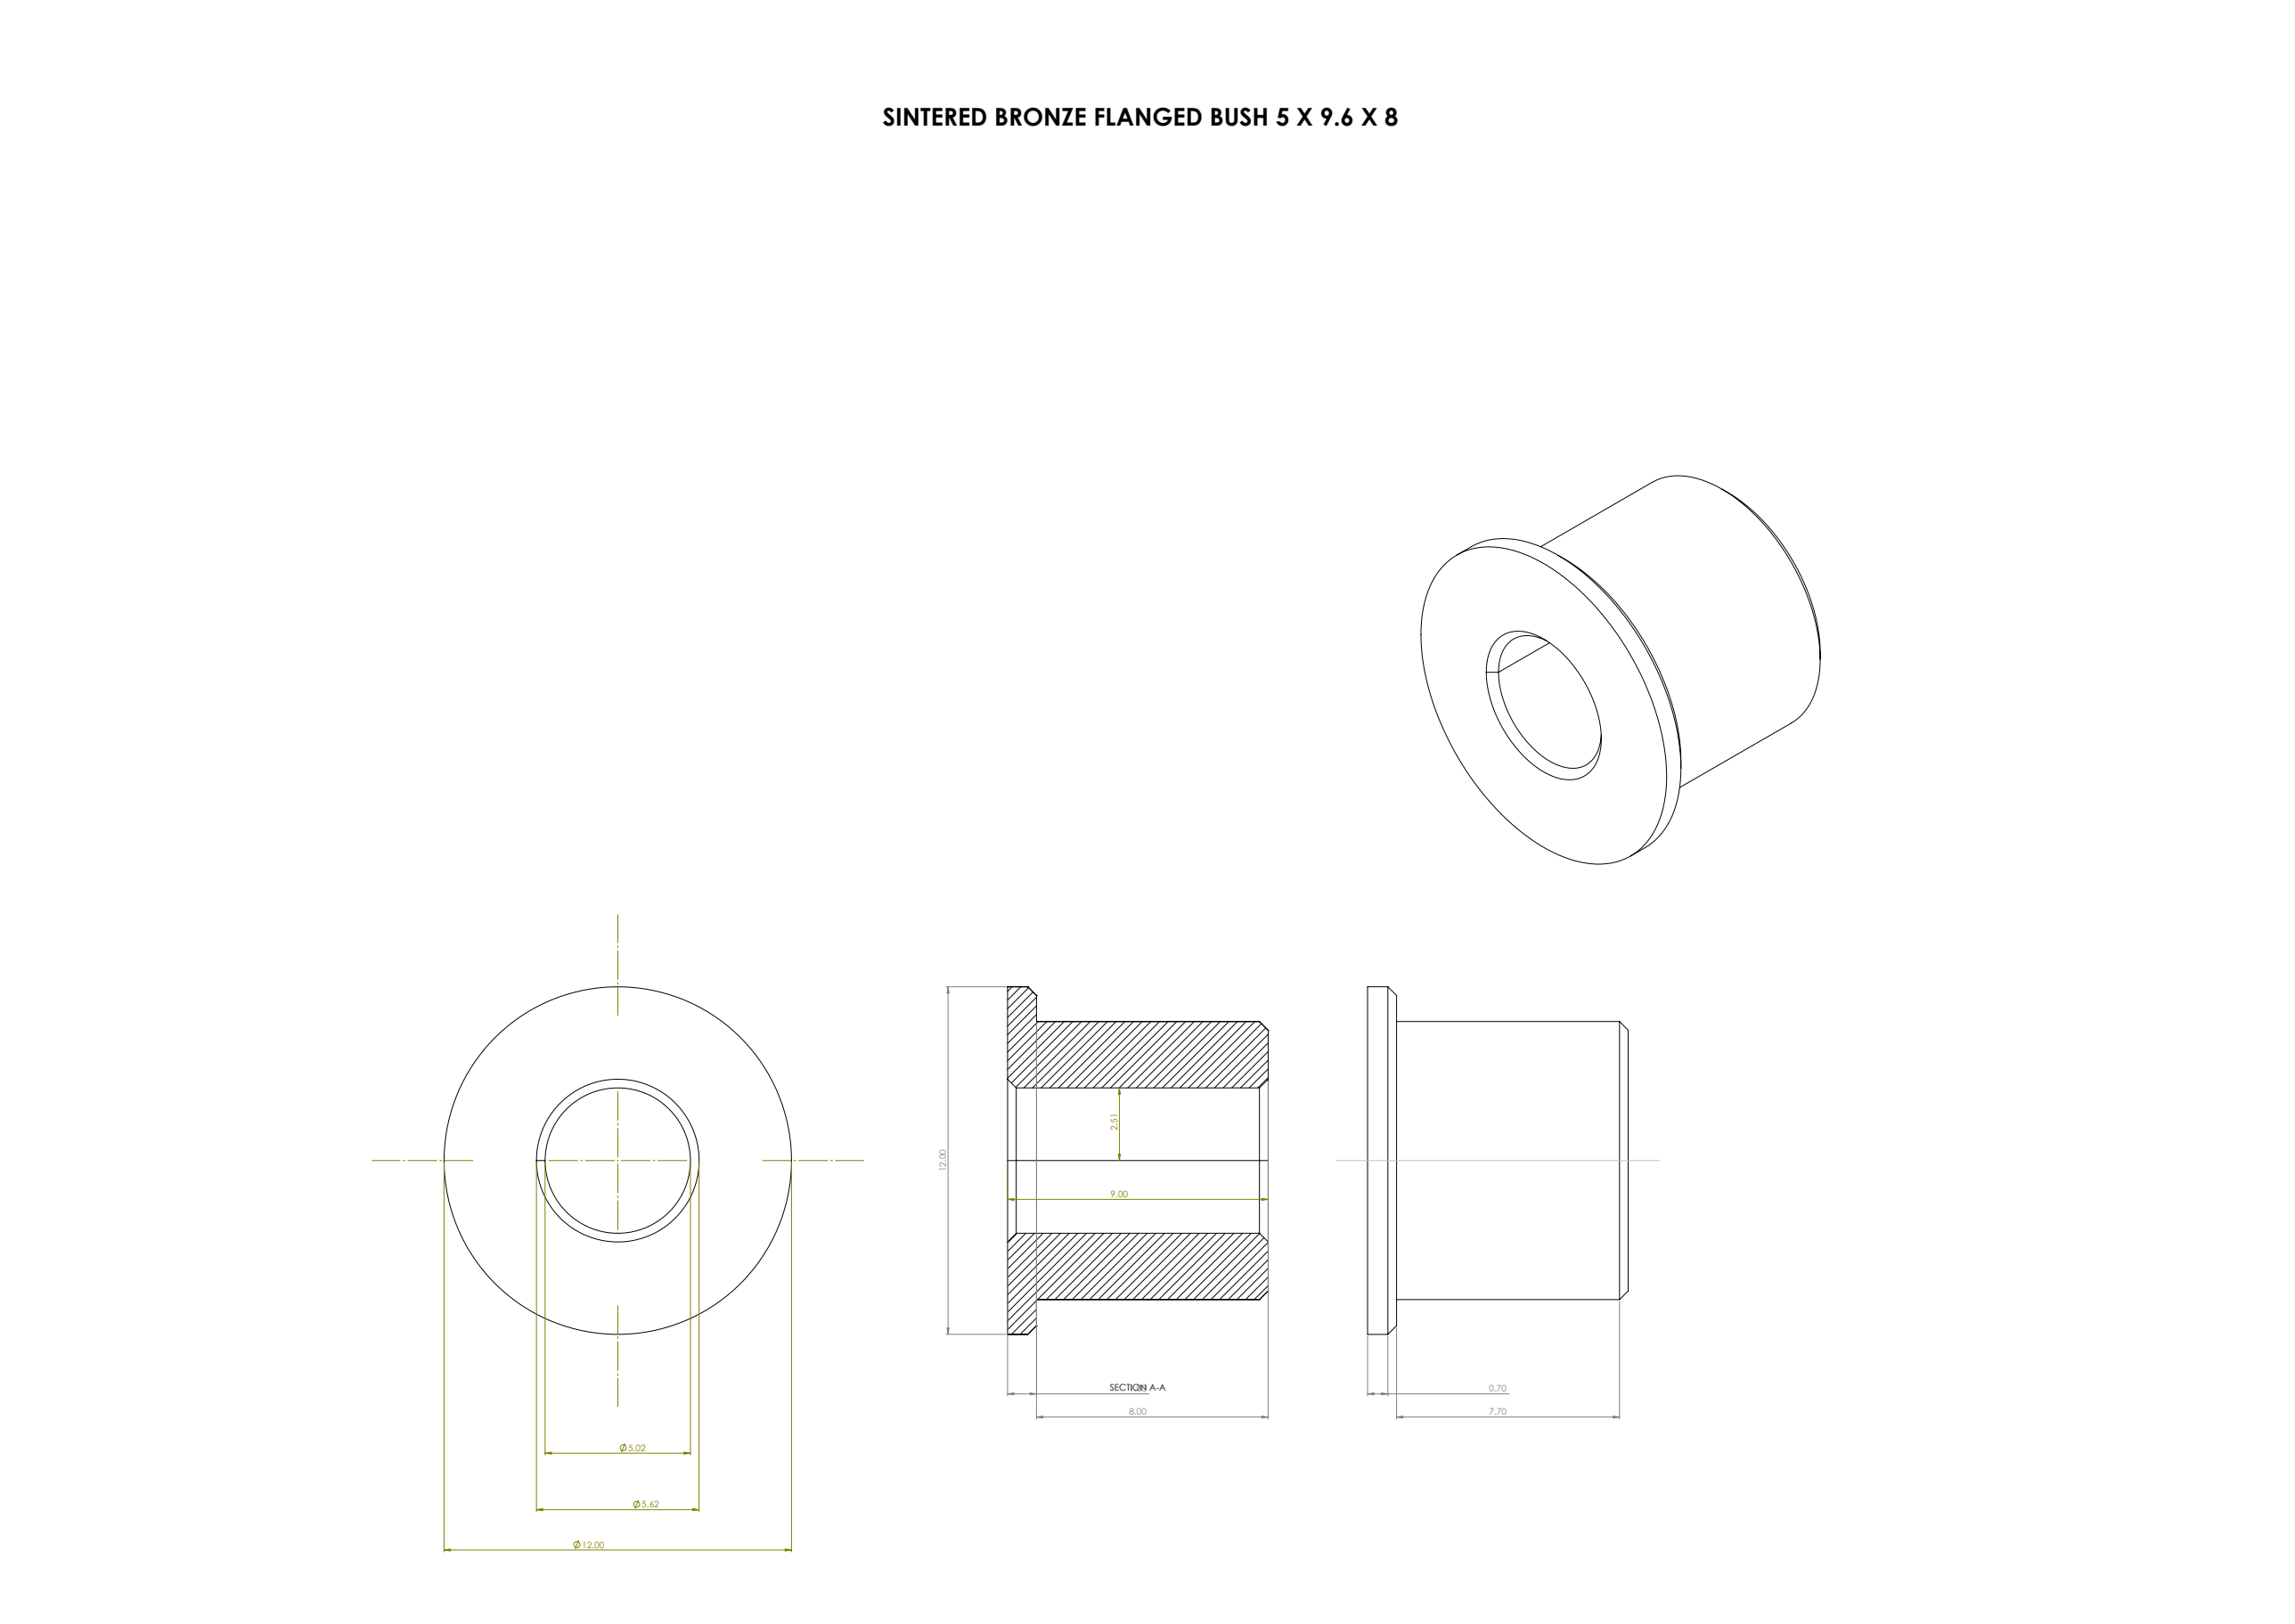
ISO-10303-21;
HEADER;
/* Generated by software containing ST-Developer
 * from STEP Tools, Inc. (www.steptools.com) 
 */

FILE_DESCRIPTION(
/* description */ (''),
/* implementation_level */ '2;1');

FILE_NAME(
/* name */ 'Sintered Bronze Flanged Bush 5 x 9.6 x 8.step',
/* time_stamp */ '2026-10-05T09:57:53+05:00',
/* author */ (''),
/* organization */ (''),
/* preprocessor_version */ 'ST-DEVELOPER v20.2',
/* originating_system */ 'Autodesk Translation Framework v15.15.0.0',
/* authorisation */ '');

FILE_SCHEMA (('AUTOMOTIVE_DESIGN { 1 0 10303 214 3 1 1 }'));
ENDSEC;

DATA;
#10=MECHANICAL_DESIGN_GEOMETRIC_PRESENTATION_REPRESENTATION('',(#557),#113984);
#521=SHAPE_REPRESENTATION_RELATIONSHIP('SRR','None',#114058,#539);
#539=ADVANCED_BREP_SHAPE_REPRESENTATION('',(#575),#113972);
#557=STYLED_ITEM('',(#114296),#575);
#575=MANIFOLD_SOLID_BREP('Sintered Bronze Flanged Bush 5 x 9.6 x 8',#60398);
#700=CYLINDRICAL_SURFACE('',#62383,4.8);
#701=CYLINDRICAL_SURFACE('',#62389,6.);
#702=CYLINDRICAL_SURFACE('',#62395,2.51000000000001);
#922=CONICAL_SURFACE('',#62376,2.66000000000002,0.785398163397434);
#923=CONICAL_SURFACE('',#62381,4.65,0.785398163397463);
#924=CONICAL_SURFACE('',#62387,5.85000000000001,0.785398163397434);
#925=CONICAL_SURFACE('',#62393,2.66000000000002,0.785398163397434);
#1234=CIRCLE('',#62377,2.51000000000001);
#1235=CIRCLE('',#62378,2.81000000000001);
#1236=CIRCLE('',#62380,4.49999999999999);
#1237=CIRCLE('',#62382,4.8);
#1238=CIRCLE('',#62384,4.8);
#1239=CIRCLE('',#62386,5.7);
#1240=CIRCLE('',#62388,6.);
#1241=CIRCLE('',#62390,6.);
#1242=CIRCLE('',#62392,2.81000000000001);
#1243=CIRCLE('',#62394,2.51000000000001);
#1838=FACE_BOUND('',#9788,.T.);
#1839=FACE_BOUND('',#9792,.T.);
#1840=FACE_BOUND('',#9796,.T.);
#3183=PLANE('',#62379);
#3184=PLANE('',#62385);
#3185=PLANE('',#62391);
#6223=FACE_OUTER_BOUND('',#9786,.T.);
#6224=FACE_OUTER_BOUND('',#9787,.T.);
#6225=FACE_OUTER_BOUND('',#9789,.T.);
#6226=FACE_OUTER_BOUND('',#9790,.T.);
#6227=FACE_OUTER_BOUND('',#9791,.T.);
#6228=FACE_OUTER_BOUND('',#9793,.T.);
#6229=FACE_OUTER_BOUND('',#9794,.T.);
#6230=FACE_OUTER_BOUND('',#9795,.T.);
#6231=FACE_OUTER_BOUND('',#9797,.T.);
#6232=FACE_OUTER_BOUND('',#9798,.T.);
#9786=EDGE_LOOP('',(#50399,#50400,#50401,#50402));
#9787=EDGE_LOOP('',(#50403));
#9788=EDGE_LOOP('',(#50404));
#9789=EDGE_LOOP('',(#50405,#50406,#50407,#50408));
#9790=EDGE_LOOP('',(#50409,#50410,#50411,#50412));
#9791=EDGE_LOOP('',(#50413));
#9792=EDGE_LOOP('',(#50414));
#9793=EDGE_LOOP('',(#50415,#50416,#50417,#50418));
#9794=EDGE_LOOP('',(#50419,#50420,#50421,#50422));
#9795=EDGE_LOOP('',(#50423));
#9796=EDGE_LOOP('',(#50424));
#9797=EDGE_LOOP('',(#50425,#50426,#50427,#50428));
#9798=EDGE_LOOP('',(#50429,#50430,#50431,#50432));
#14630=LINE('',#98912,#20664);
#14631=LINE('',#98920,#20665);
#14632=LINE('',#98924,#20666);
#14633=LINE('',#98931,#20667);
#14634=LINE('',#98935,#20668);
#14635=LINE('',#98941,#20669);
#14636=LINE('',#98944,#20670);
#20664=VECTOR('',#71068,2.66000000000002);
#20665=VECTOR('',#71079,4.65);
#20666=VECTOR('',#71084,4.8);
#20667=VECTOR('',#71093,5.85000000000001);
#20668=VECTOR('',#71098,6.);
#20669=VECTOR('',#71105,2.66000000000002);
#20670=VECTOR('',#71110,2.51000000000001);
#28381=VERTEX_POINT('',#98909);
#28382=VERTEX_POINT('',#98911);
#28383=VERTEX_POINT('',#98915);
#28384=VERTEX_POINT('',#98918);
#28385=VERTEX_POINT('',#98922);
#28386=VERTEX_POINT('',#98926);
#28387=VERTEX_POINT('',#98929);
#28388=VERTEX_POINT('',#98933);
#28389=VERTEX_POINT('',#98937);
#28390=VERTEX_POINT('',#98940);
#36032=EDGE_CURVE('',#28381,#28381,#1234,.T.);
#36033=EDGE_CURVE('',#28381,#28382,#14630,.T.);
#36034=EDGE_CURVE('',#28382,#28382,#1235,.T.);
#36035=EDGE_CURVE('',#28383,#28383,#1236,.T.);
#36036=EDGE_CURVE('',#28384,#28384,#1237,.T.);
#36037=EDGE_CURVE('',#28384,#28383,#14631,.T.);
#36038=EDGE_CURVE('',#28385,#28385,#1238,.T.);
#36039=EDGE_CURVE('',#28385,#28384,#14632,.T.);
#36040=EDGE_CURVE('',#28386,#28386,#1239,.T.);
#36041=EDGE_CURVE('',#28387,#28387,#1240,.T.);
#36042=EDGE_CURVE('',#28387,#28386,#14633,.T.);
#36043=EDGE_CURVE('',#28388,#28388,#1241,.T.);
#36044=EDGE_CURVE('',#28388,#28387,#14634,.T.);
#36045=EDGE_CURVE('',#28389,#28389,#1242,.T.);
#36046=EDGE_CURVE('',#28389,#28390,#14635,.T.);
#36047=EDGE_CURVE('',#28390,#28390,#1243,.T.);
#36048=EDGE_CURVE('',#28390,#28381,#14636,.T.);
#50399=ORIENTED_EDGE('',*,*,#36032,.T.);
#50400=ORIENTED_EDGE('',*,*,#36033,.T.);
#50401=ORIENTED_EDGE('',*,*,#36034,.F.);
#50402=ORIENTED_EDGE('',*,*,#36033,.F.);
#50403=ORIENTED_EDGE('',*,*,#36035,.F.);
#50404=ORIENTED_EDGE('',*,*,#36034,.T.);
#50405=ORIENTED_EDGE('',*,*,#36036,.F.);
#50406=ORIENTED_EDGE('',*,*,#36037,.T.);
#50407=ORIENTED_EDGE('',*,*,#36035,.T.);
#50408=ORIENTED_EDGE('',*,*,#36037,.F.);
#50409=ORIENTED_EDGE('',*,*,#36038,.F.);
#50410=ORIENTED_EDGE('',*,*,#36039,.T.);
#50411=ORIENTED_EDGE('',*,*,#36036,.T.);
#50412=ORIENTED_EDGE('',*,*,#36039,.F.);
#50413=ORIENTED_EDGE('',*,*,#36040,.F.);
#50414=ORIENTED_EDGE('',*,*,#36038,.T.);
#50415=ORIENTED_EDGE('',*,*,#36041,.F.);
#50416=ORIENTED_EDGE('',*,*,#36042,.T.);
#50417=ORIENTED_EDGE('',*,*,#36040,.T.);
#50418=ORIENTED_EDGE('',*,*,#36042,.F.);
#50419=ORIENTED_EDGE('',*,*,#36043,.F.);
#50420=ORIENTED_EDGE('',*,*,#36044,.T.);
#50421=ORIENTED_EDGE('',*,*,#36041,.T.);
#50422=ORIENTED_EDGE('',*,*,#36044,.F.);
#50423=ORIENTED_EDGE('',*,*,#36043,.T.);
#50424=ORIENTED_EDGE('',*,*,#36045,.F.);
#50425=ORIENTED_EDGE('',*,*,#36045,.T.);
#50426=ORIENTED_EDGE('',*,*,#36046,.T.);
#50427=ORIENTED_EDGE('',*,*,#36047,.F.);
#50428=ORIENTED_EDGE('',*,*,#36046,.F.);
#50429=ORIENTED_EDGE('',*,*,#36047,.T.);
#50430=ORIENTED_EDGE('',*,*,#36048,.T.);
#50431=ORIENTED_EDGE('',*,*,#36032,.F.);
#50432=ORIENTED_EDGE('',*,*,#36048,.F.);
#59323=ADVANCED_FACE('',(#6223),#922,.F.);
#59324=ADVANCED_FACE('',(#6224,#1838),#3183,.T.);
#59325=ADVANCED_FACE('',(#6225),#923,.T.);
#59326=ADVANCED_FACE('',(#6226),#700,.T.);
#59327=ADVANCED_FACE('',(#6227,#1839),#3184,.T.);
#59328=ADVANCED_FACE('',(#6228),#924,.T.);
#59329=ADVANCED_FACE('',(#6229),#701,.T.);
#59330=ADVANCED_FACE('',(#6230,#1840),#3185,.T.);
#59331=ADVANCED_FACE('',(#6231),#925,.F.);
#59332=ADVANCED_FACE('',(#6232),#702,.F.);
#60398=CLOSED_SHELL('',(#59323,#59324,#59325,#59326,#59327,#59328,#59329,
#59330,#59331,#59332));
#62375=AXIS2_PLACEMENT_3D('',#98907,#71062,#71063);
#62376=AXIS2_PLACEMENT_3D('',#98908,#71064,#71065);
#62377=AXIS2_PLACEMENT_3D('',#98910,#71066,#71067);
#62378=AXIS2_PLACEMENT_3D('',#98913,#71069,#71070);
#62379=AXIS2_PLACEMENT_3D('',#98914,#71071,#71072);
#62380=AXIS2_PLACEMENT_3D('',#98916,#71073,#71074);
#62381=AXIS2_PLACEMENT_3D('',#98917,#71075,#71076);
#62382=AXIS2_PLACEMENT_3D('',#98919,#71077,#71078);
#62383=AXIS2_PLACEMENT_3D('',#98921,#71080,#71081);
#62384=AXIS2_PLACEMENT_3D('',#98923,#71082,#71083);
#62385=AXIS2_PLACEMENT_3D('',#98925,#71085,#71086);
#62386=AXIS2_PLACEMENT_3D('',#98927,#71087,#71088);
#62387=AXIS2_PLACEMENT_3D('',#98928,#71089,#71090);
#62388=AXIS2_PLACEMENT_3D('',#98930,#71091,#71092);
#62389=AXIS2_PLACEMENT_3D('',#98932,#71094,#71095);
#62390=AXIS2_PLACEMENT_3D('',#98934,#71096,#71097);
#62391=AXIS2_PLACEMENT_3D('',#98936,#71099,#71100);
#62392=AXIS2_PLACEMENT_3D('',#98938,#71101,#71102);
#62393=AXIS2_PLACEMENT_3D('',#98939,#71103,#71104);
#62394=AXIS2_PLACEMENT_3D('',#98942,#71106,#71107);
#62395=AXIS2_PLACEMENT_3D('',#98943,#71108,#71109);
#71062=DIRECTION('axis',(0.,0.,1.));
#71063=DIRECTION('refdir',(1.,0.,0.));
#71064=DIRECTION('center_axis',(0.,0.,-1.));
#71065=DIRECTION('ref_axis',(1.,0.,0.));
#71066=DIRECTION('center_axis',(0.,0.,1.));
#71067=DIRECTION('ref_axis',(1.,0.,0.));
#71068=DIRECTION('',(-0.707106781186537,-8.6595605623548E-17,-0.707106781186558));
#71069=DIRECTION('center_axis',(0.,0.,1.));
#71070=DIRECTION('ref_axis',(1.,0.,0.));
#71071=DIRECTION('center_axis',(0.,0.,-1.));
#71072=DIRECTION('ref_axis',(-1.,0.,0.));
#71073=DIRECTION('center_axis',(0.,0.,1.));
#71074=DIRECTION('ref_axis',(1.,0.,0.));
#71075=DIRECTION('center_axis',(0.,0.,1.));
#71076=DIRECTION('ref_axis',(1.,0.,0.));
#71077=DIRECTION('center_axis',(0.,0.,1.));
#71078=DIRECTION('ref_axis',(1.,0.,0.));
#71079=DIRECTION('',(0.707106781186558,8.65956056235506E-17,-0.707106781186537));
#71080=DIRECTION('center_axis',(0.,0.,1.));
#71081=DIRECTION('ref_axis',(1.,0.,0.));
#71082=DIRECTION('center_axis',(0.,0.,1.));
#71083=DIRECTION('ref_axis',(1.,0.,0.));
#71084=DIRECTION('',(0.,0.,-1.));
#71085=DIRECTION('center_axis',(0.,0.,-1.));
#71086=DIRECTION('ref_axis',(-1.,0.,0.));
#71087=DIRECTION('center_axis',(0.,0.,1.));
#71088=DIRECTION('ref_axis',(1.,0.,0.));
#71089=DIRECTION('center_axis',(0.,0.,1.));
#71090=DIRECTION('ref_axis',(1.,0.,0.));
#71091=DIRECTION('center_axis',(0.,0.,1.));
#71092=DIRECTION('ref_axis',(1.,0.,0.));
#71093=DIRECTION('',(0.707106781186537,8.6595605623548E-17,-0.707106781186558));
#71094=DIRECTION('center_axis',(0.,0.,1.));
#71095=DIRECTION('ref_axis',(1.,0.,0.));
#71096=DIRECTION('center_axis',(0.,0.,1.));
#71097=DIRECTION('ref_axis',(1.,0.,0.));
#71098=DIRECTION('',(0.,0.,-1.));
#71099=DIRECTION('center_axis',(0.,0.,1.));
#71100=DIRECTION('ref_axis',(1.,0.,0.));
#71101=DIRECTION('center_axis',(0.,0.,1.));
#71102=DIRECTION('ref_axis',(1.,0.,0.));
#71103=DIRECTION('center_axis',(0.,0.,1.));
#71104=DIRECTION('ref_axis',(1.,0.,0.));
#71105=DIRECTION('',(0.707106781186537,8.6595605623548E-17,-0.707106781186558));
#71106=DIRECTION('center_axis',(0.,0.,1.));
#71107=DIRECTION('ref_axis',(1.,0.,0.));
#71108=DIRECTION('center_axis',(0.,0.,1.));
#71109=DIRECTION('ref_axis',(1.,0.,0.));
#71110=DIRECTION('',(0.,0.,-1.));
#98907=CARTESIAN_POINT('',(0.,0.,0.));
#98908=CARTESIAN_POINT('Origin',(110.,18.,40.65));
#98909=CARTESIAN_POINT('',(107.49,18.,40.8));
#98910=CARTESIAN_POINT('Origin',(110.,18.,40.8));
#98911=CARTESIAN_POINT('',(107.19,18.,40.5));
#98912=CARTESIAN_POINT('',(107.34,18.,40.65));
#98913=CARTESIAN_POINT('Origin',(110.,18.,40.5));
#98914=CARTESIAN_POINT('Origin',(114.5,18.,40.5));
#98915=CARTESIAN_POINT('',(105.5,18.,40.5));
#98916=CARTESIAN_POINT('Origin',(110.,18.,40.5));
#98917=CARTESIAN_POINT('Origin',(110.,18.,40.65));
#98918=CARTESIAN_POINT('',(105.2,18.,40.8));
#98919=CARTESIAN_POINT('Origin',(110.,18.,40.8));
#98920=CARTESIAN_POINT('',(105.35,18.,40.65));
#98921=CARTESIAN_POINT('Origin',(110.,18.,44.65));
#98922=CARTESIAN_POINT('',(105.2,18.,48.5));
#98923=CARTESIAN_POINT('Origin',(110.,18.,48.5));
#98924=CARTESIAN_POINT('',(105.2,18.,44.65));
#98925=CARTESIAN_POINT('Origin',(115.7,18.,48.5));
#98926=CARTESIAN_POINT('',(104.3,18.,48.5));
#98927=CARTESIAN_POINT('Origin',(110.,18.,48.5));
#98928=CARTESIAN_POINT('Origin',(110.,18.,48.65));
#98929=CARTESIAN_POINT('',(104.,18.,48.8));
#98930=CARTESIAN_POINT('Origin',(110.,18.,48.8));
#98931=CARTESIAN_POINT('',(104.15,18.,48.65));
#98932=CARTESIAN_POINT('Origin',(110.,18.,49.15));
#98933=CARTESIAN_POINT('',(104.,18.,49.5));
#98934=CARTESIAN_POINT('Origin',(110.,18.,49.5));
#98935=CARTESIAN_POINT('',(104.,18.,49.15));
#98936=CARTESIAN_POINT('Origin',(112.81,18.,49.5));
#98937=CARTESIAN_POINT('',(107.19,18.,49.5));
#98938=CARTESIAN_POINT('Origin',(110.,18.,49.5));
#98939=CARTESIAN_POINT('Origin',(110.,18.,49.35));
#98940=CARTESIAN_POINT('',(107.49,18.,49.2));
#98941=CARTESIAN_POINT('',(107.34,18.,49.35));
#98942=CARTESIAN_POINT('Origin',(110.,18.,49.2));
#98943=CARTESIAN_POINT('Origin',(110.,18.,45.));
#98944=CARTESIAN_POINT('',(107.49,18.,45.));
#113952=UNCERTAINTY_MEASURE_WITH_UNIT(LENGTH_MEASURE(0.01),#113985,
'DISTANCE_ACCURACY_VALUE',
'Maximum model space distance between geometric entities at asserted c
onnectivities');
#113964=UNCERTAINTY_MEASURE_WITH_UNIT(LENGTH_MEASURE(0.01),#113985,
'DISTANCE_ACCURACY_VALUE',
'Maximum model space distance between geometric entities at asserted c
onnectivities');
#113972=(
GEOMETRIC_REPRESENTATION_CONTEXT(3)
GLOBAL_UNCERTAINTY_ASSIGNED_CONTEXT((#113952))
GLOBAL_UNIT_ASSIGNED_CONTEXT((#113985,#113987,#113988))
REPRESENTATION_CONTEXT('','3D')
);
#113984=(
GEOMETRIC_REPRESENTATION_CONTEXT(3)
GLOBAL_UNCERTAINTY_ASSIGNED_CONTEXT((#113964))
GLOBAL_UNIT_ASSIGNED_CONTEXT((#113985,#113987,#113988))
REPRESENTATION_CONTEXT('','3D')
);
#113985=(
LENGTH_UNIT()
NAMED_UNIT(*)
SI_UNIT(.MILLI.,.METRE.)
);
#113987=(
NAMED_UNIT(*)
PLANE_ANGLE_UNIT()
SI_UNIT($,.RADIAN.)
);
#113988=(
NAMED_UNIT(*)
SI_UNIT($,.STERADIAN.)
SOLID_ANGLE_UNIT()
);
#113996=SHAPE_DEFINITION_REPRESENTATION(#114015,#114058);
#114015=PRODUCT_DEFINITION_SHAPE('',$,#114078);
#114058=SHAPE_REPRESENTATION('',(#62375),#113972);
#114070=PRODUCT_DEFINITION_CONTEXT('part definition',#114129,'design');
#114078=PRODUCT_DEFINITION('2026-10-05-09-49-27-315',
'Sintered Bronze Flanged Bush 5 x 9.6 x 8',#114097,#114070);
#114097=PRODUCT_DEFINITION_FORMATION('',$,#114138);
#114129=APPLICATION_CONTEXT(
'Core Data for Automotive Mechanical Design Process');
#114130=PRODUCT_CONTEXT('part definition',#114129,'mechanical');
#114138=PRODUCT('2026-10-05-09-49-27-315',
'Sintered Bronze Flanged Bush 5 x 9.6 x 8',$,(#114130));
#114290=COLOUR_RGB('Light Blue',0.38,0.62,0.78);
#114291=FILL_AREA_STYLE_COLOUR('',#114290);
#114292=FILL_AREA_STYLE('',(#114291));
#114293=SURFACE_STYLE_FILL_AREA(#114292);
#114294=SURFACE_SIDE_STYLE('',(#114293));
#114295=SURFACE_STYLE_USAGE(.BOTH.,#114294);
#114296=PRESENTATION_STYLE_ASSIGNMENT((#114295));
ENDSEC;
END-ISO-10303-21;
